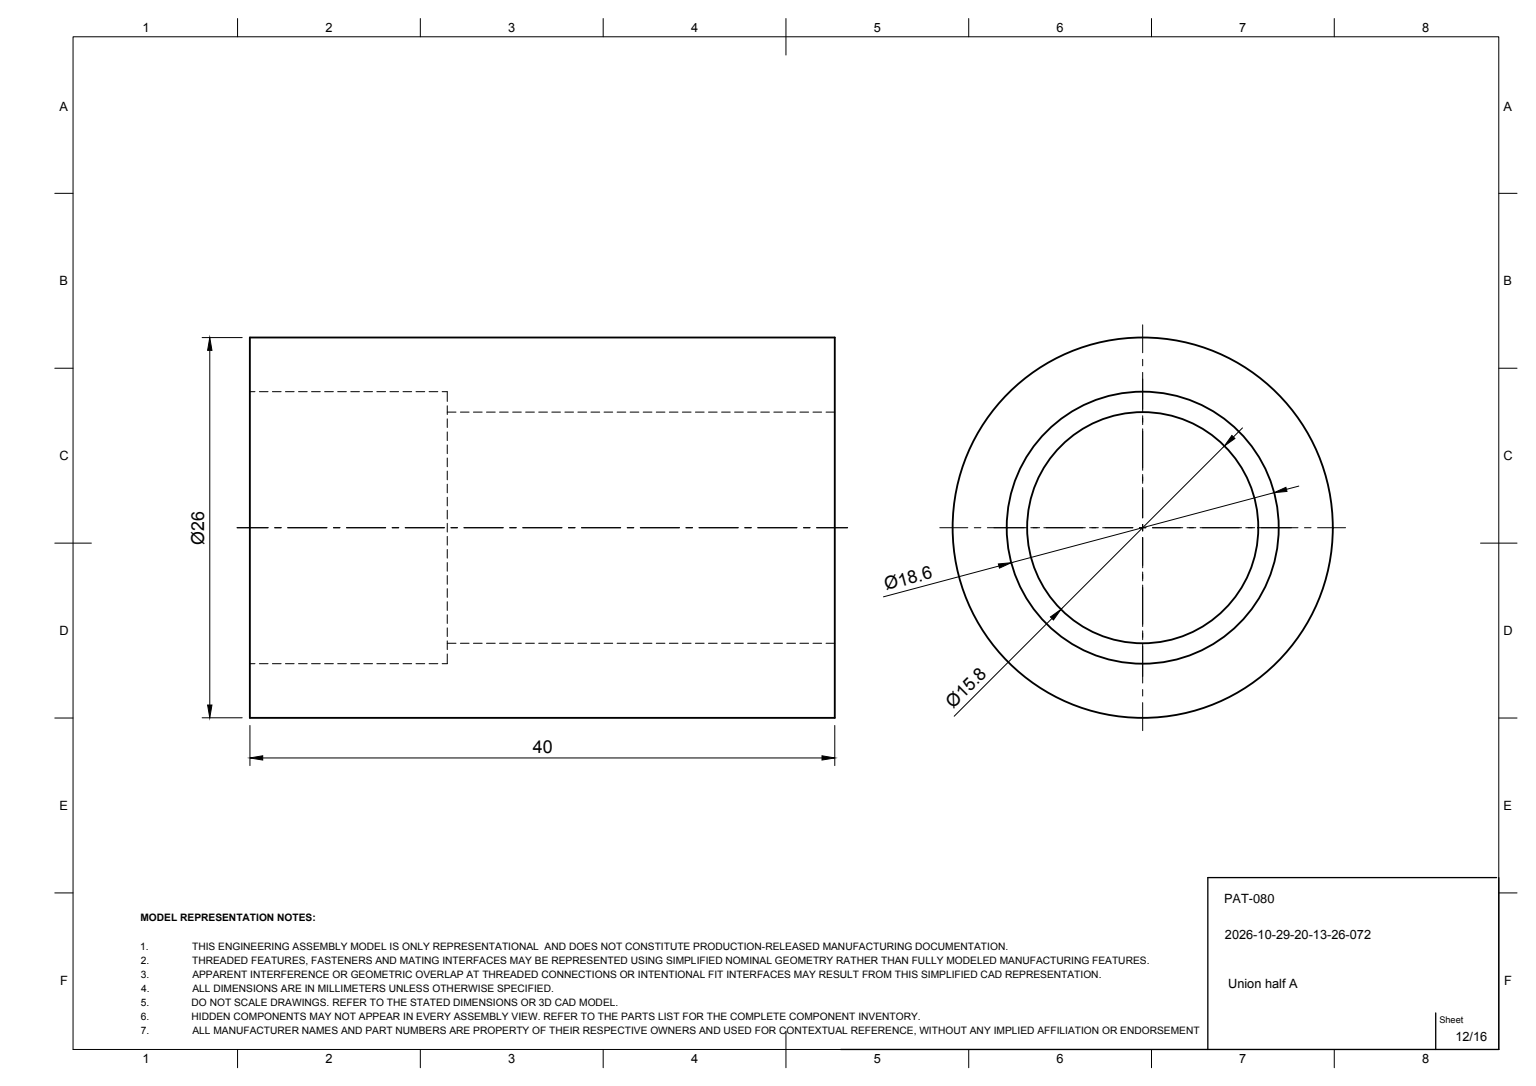
ISO-10303-21;
HEADER;
/* Generated by software containing ST-Developer
 * from STEP Tools, Inc. (www.steptools.com) 
 */

FILE_DESCRIPTION(
/* description */ ('PAT-080'),
/* implementation_level */ '2;1');

FILE_NAME(
/* name */ 'Union half A.step',
/* time_stamp */ '2026-10-29T20:13:47-07:00',
/* author */ (''),
/* organization */ (''),
/* preprocessor_version */ 'ST-DEVELOPER v20.2',
/* originating_system */ 'Autodesk Translation Framework v15.17.0.0',
/* authorisation */ '');

FILE_SCHEMA (('AUTOMOTIVE_DESIGN { 1 0 10303 214 3 1 1 }'));
ENDSEC;

DATA;
#10=MECHANICAL_DESIGN_GEOMETRIC_PRESENTATION_REPRESENTATION('',(#254),#6878);
#216=SHAPE_REPRESENTATION_RELATIONSHIP('SRR','None',#6972,#235);
#235=ADVANCED_BREP_SHAPE_REPRESENTATION('',(#273),#6867);
#254=STYLED_ITEM('',(#7143),#273);
#273=MANIFOLD_SOLID_BREP('Body1',#3870);
#312=FACE_BOUND('',#862,.T.);
#313=FACE_BOUND('',#863,.T.);
#314=FACE_BOUND('',#864,.T.);
#315=FACE_BOUND('',#865,.T.);
#316=FACE_BOUND('',#866,.T.);
#317=FACE_BOUND('',#871,.T.);
#318=FACE_BOUND('',#872,.T.);
#319=FACE_BOUND('',#873,.T.);
#320=FACE_BOUND('',#874,.T.);
#321=FACE_BOUND('',#875,.T.);
#322=FACE_BOUND('',#877,.T.);
#430=PLANE('',#4270);
#431=PLANE('',#4280);
#432=PLANE('',#4281);
#600=FACE_OUTER_BOUND('',#857,.T.);
#601=FACE_OUTER_BOUND('',#858,.T.);
#602=FACE_OUTER_BOUND('',#859,.T.);
#603=FACE_OUTER_BOUND('',#860,.T.);
#604=FACE_OUTER_BOUND('',#861,.T.);
#605=FACE_OUTER_BOUND('',#867,.T.);
#606=FACE_OUTER_BOUND('',#868,.T.);
#607=FACE_OUTER_BOUND('',#869,.T.);
#608=FACE_OUTER_BOUND('',#870,.T.);
#609=FACE_OUTER_BOUND('',#876,.T.);
#857=EDGE_LOOP('',(#3082,#3083,#3084,#3085));
#858=EDGE_LOOP('',(#3086,#3087,#3088,#3089));
#859=EDGE_LOOP('',(#3090,#3091,#3092,#3093));
#860=EDGE_LOOP('',(#3094,#3095,#3096,#3097));
#861=EDGE_LOOP('',(#3098));
#862=EDGE_LOOP('',(#3099));
#863=EDGE_LOOP('',(#3100));
#864=EDGE_LOOP('',(#3101));
#865=EDGE_LOOP('',(#3102));
#866=EDGE_LOOP('',(#3103));
#867=EDGE_LOOP('',(#3104,#3105,#3106,#3107));
#868=EDGE_LOOP('',(#3108,#3109,#3110,#3111));
#869=EDGE_LOOP('',(#3112,#3113,#3114,#3115));
#870=EDGE_LOOP('',(#3116));
#871=EDGE_LOOP('',(#3117));
#872=EDGE_LOOP('',(#3118));
#873=EDGE_LOOP('',(#3119));
#874=EDGE_LOOP('',(#3120));
#875=EDGE_LOOP('',(#3121));
#876=EDGE_LOOP('',(#3122));
#877=EDGE_LOOP('',(#3123));
#1211=LINE('',#6238,#1526);
#1212=LINE('',#6244,#1527);
#1213=LINE('',#6250,#1528);
#1214=LINE('',#6256,#1529);
#1215=LINE('',#6266,#1530);
#1216=LINE('',#6271,#1531);
#1217=LINE('',#6275,#1532);
#1526=VECTOR('',#5049,0.44);
#1527=VECTOR('',#5056,0.44);
#1528=VECTOR('',#5063,0.44);
#1529=VECTOR('',#5070,0.44);
#1530=VECTOR('',#5083,3.5);
#1531=VECTOR('',#5088,0.79);
#1532=VECTOR('',#5093,1.5);
#1712=CIRCLE('',#4259,0.44);
#1713=CIRCLE('',#4260,0.44);
#1714=CIRCLE('',#4262,0.44);
#1715=CIRCLE('',#4263,0.44);
#1716=CIRCLE('',#4265,0.44);
#1717=CIRCLE('',#4266,0.44);
#1718=CIRCLE('',#4268,0.44);
#1719=CIRCLE('',#4269,0.44);
#1720=CIRCLE('',#4271,3.5);
#1721=CIRCLE('',#4272,1.5);
#1722=CIRCLE('',#4274,3.5);
#1723=CIRCLE('',#4276,0.79);
#1724=CIRCLE('',#4277,0.79);
#1725=CIRCLE('',#4279,1.5);
#1968=VERTEX_POINT('',#6235);
#1969=VERTEX_POINT('',#6237);
#1970=VERTEX_POINT('',#6241);
#1971=VERTEX_POINT('',#6243);
#1972=VERTEX_POINT('',#6247);
#1973=VERTEX_POINT('',#6249);
#1974=VERTEX_POINT('',#6253);
#1975=VERTEX_POINT('',#6255);
#1976=VERTEX_POINT('',#6259);
#1977=VERTEX_POINT('',#6261);
#1978=VERTEX_POINT('',#6264);
#1979=VERTEX_POINT('',#6268);
#1980=VERTEX_POINT('',#6270);
#1981=VERTEX_POINT('',#6274);
#2364=EDGE_CURVE('',#1968,#1968,#1712,.T.);
#2365=EDGE_CURVE('',#1968,#1969,#1211,.T.);
#2366=EDGE_CURVE('',#1969,#1969,#1713,.T.);
#2367=EDGE_CURVE('',#1970,#1970,#1714,.T.);
#2368=EDGE_CURVE('',#1970,#1971,#1212,.T.);
#2369=EDGE_CURVE('',#1971,#1971,#1715,.T.);
#2370=EDGE_CURVE('',#1972,#1972,#1716,.T.);
#2371=EDGE_CURVE('',#1972,#1973,#1213,.T.);
#2372=EDGE_CURVE('',#1973,#1973,#1717,.T.);
#2373=EDGE_CURVE('',#1974,#1974,#1718,.T.);
#2374=EDGE_CURVE('',#1974,#1975,#1214,.T.);
#2375=EDGE_CURVE('',#1975,#1975,#1719,.T.);
#2376=EDGE_CURVE('',#1976,#1976,#1720,.T.);
#2377=EDGE_CURVE('',#1977,#1977,#1721,.T.);
#2378=EDGE_CURVE('',#1978,#1978,#1722,.T.);
#2379=EDGE_CURVE('',#1978,#1976,#1215,.T.);
#2380=EDGE_CURVE('',#1979,#1979,#1723,.T.);
#2381=EDGE_CURVE('',#1979,#1980,#1216,.T.);
#2382=EDGE_CURVE('',#1980,#1980,#1724,.T.);
#2383=EDGE_CURVE('',#1977,#1981,#1217,.T.);
#2384=EDGE_CURVE('',#1981,#1981,#1725,.T.);
#3082=ORIENTED_EDGE('',*,*,#2364,.F.);
#3083=ORIENTED_EDGE('',*,*,#2365,.T.);
#3084=ORIENTED_EDGE('',*,*,#2366,.F.);
#3085=ORIENTED_EDGE('',*,*,#2365,.F.);
#3086=ORIENTED_EDGE('',*,*,#2367,.F.);
#3087=ORIENTED_EDGE('',*,*,#2368,.T.);
#3088=ORIENTED_EDGE('',*,*,#2369,.F.);
#3089=ORIENTED_EDGE('',*,*,#2368,.F.);
#3090=ORIENTED_EDGE('',*,*,#2370,.F.);
#3091=ORIENTED_EDGE('',*,*,#2371,.T.);
#3092=ORIENTED_EDGE('',*,*,#2372,.F.);
#3093=ORIENTED_EDGE('',*,*,#2371,.F.);
#3094=ORIENTED_EDGE('',*,*,#2373,.F.);
#3095=ORIENTED_EDGE('',*,*,#2374,.T.);
#3096=ORIENTED_EDGE('',*,*,#2375,.F.);
#3097=ORIENTED_EDGE('',*,*,#2374,.F.);
#3098=ORIENTED_EDGE('',*,*,#2376,.F.);
#3099=ORIENTED_EDGE('',*,*,#2377,.F.);
#3100=ORIENTED_EDGE('',*,*,#2373,.T.);
#3101=ORIENTED_EDGE('',*,*,#2370,.T.);
#3102=ORIENTED_EDGE('',*,*,#2367,.T.);
#3103=ORIENTED_EDGE('',*,*,#2364,.T.);
#3104=ORIENTED_EDGE('',*,*,#2378,.F.);
#3105=ORIENTED_EDGE('',*,*,#2379,.T.);
#3106=ORIENTED_EDGE('',*,*,#2376,.T.);
#3107=ORIENTED_EDGE('',*,*,#2379,.F.);
#3108=ORIENTED_EDGE('',*,*,#2380,.F.);
#3109=ORIENTED_EDGE('',*,*,#2381,.T.);
#3110=ORIENTED_EDGE('',*,*,#2382,.T.);
#3111=ORIENTED_EDGE('',*,*,#2381,.F.);
#3112=ORIENTED_EDGE('',*,*,#2377,.T.);
#3113=ORIENTED_EDGE('',*,*,#2383,.T.);
#3114=ORIENTED_EDGE('',*,*,#2384,.T.);
#3115=ORIENTED_EDGE('',*,*,#2383,.F.);
#3116=ORIENTED_EDGE('',*,*,#2378,.T.);
#3117=ORIENTED_EDGE('',*,*,#2380,.T.);
#3118=ORIENTED_EDGE('',*,*,#2375,.T.);
#3119=ORIENTED_EDGE('',*,*,#2372,.T.);
#3120=ORIENTED_EDGE('',*,*,#2369,.T.);
#3121=ORIENTED_EDGE('',*,*,#2366,.T.);
#3122=ORIENTED_EDGE('',*,*,#2384,.F.);
#3123=ORIENTED_EDGE('',*,*,#2382,.F.);
#3597=CYLINDRICAL_SURFACE('',#4258,0.44);
#3598=CYLINDRICAL_SURFACE('',#4261,0.44);
#3599=CYLINDRICAL_SURFACE('',#4264,0.44);
#3600=CYLINDRICAL_SURFACE('',#4267,0.44);
#3601=CYLINDRICAL_SURFACE('',#4273,3.5);
#3602=CYLINDRICAL_SURFACE('',#4275,0.79);
#3603=CYLINDRICAL_SURFACE('',#4278,1.5);
#3736=ADVANCED_FACE('',(#600),#3597,.F.);
#3737=ADVANCED_FACE('',(#601),#3598,.F.);
#3738=ADVANCED_FACE('',(#602),#3599,.F.);
#3739=ADVANCED_FACE('',(#603),#3600,.F.);
#3740=ADVANCED_FACE('',(#604,#312,#313,#314,#315,#316),#430,.F.);
#3741=ADVANCED_FACE('',(#605),#3601,.T.);
#3742=ADVANCED_FACE('',(#606),#3602,.F.);
#3743=ADVANCED_FACE('',(#607),#3603,.T.);
#3744=ADVANCED_FACE('',(#608,#317,#318,#319,#320,#321),#431,.T.);
#3745=ADVANCED_FACE('',(#609,#322),#432,.F.);
#3870=CLOSED_SHELL('',(#3736,#3737,#3738,#3739,#3740,#3741,#3742,#3743,
#3744,#3745));
#4257=AXIS2_PLACEMENT_3D('',#6233,#5043,#5044);
#4258=AXIS2_PLACEMENT_3D('',#6234,#5045,#5046);
#4259=AXIS2_PLACEMENT_3D('',#6236,#5047,#5048);
#4260=AXIS2_PLACEMENT_3D('',#6239,#5050,#5051);
#4261=AXIS2_PLACEMENT_3D('',#6240,#5052,#5053);
#4262=AXIS2_PLACEMENT_3D('',#6242,#5054,#5055);
#4263=AXIS2_PLACEMENT_3D('',#6245,#5057,#5058);
#4264=AXIS2_PLACEMENT_3D('',#6246,#5059,#5060);
#4265=AXIS2_PLACEMENT_3D('',#6248,#5061,#5062);
#4266=AXIS2_PLACEMENT_3D('',#6251,#5064,#5065);
#4267=AXIS2_PLACEMENT_3D('',#6252,#5066,#5067);
#4268=AXIS2_PLACEMENT_3D('',#6254,#5068,#5069);
#4269=AXIS2_PLACEMENT_3D('',#6257,#5071,#5072);
#4270=AXIS2_PLACEMENT_3D('',#6258,#5073,#5074);
#4271=AXIS2_PLACEMENT_3D('',#6260,#5075,#5076);
#4272=AXIS2_PLACEMENT_3D('',#6262,#5077,#5078);
#4273=AXIS2_PLACEMENT_3D('',#6263,#5079,#5080);
#4274=AXIS2_PLACEMENT_3D('',#6265,#5081,#5082);
#4275=AXIS2_PLACEMENT_3D('',#6267,#5084,#5085);
#4276=AXIS2_PLACEMENT_3D('',#6269,#5086,#5087);
#4277=AXIS2_PLACEMENT_3D('',#6272,#5089,#5090);
#4278=AXIS2_PLACEMENT_3D('',#6273,#5091,#5092);
#4279=AXIS2_PLACEMENT_3D('',#6276,#5094,#5095);
#4280=AXIS2_PLACEMENT_3D('',#6277,#5096,#5097);
#4281=AXIS2_PLACEMENT_3D('',#6278,#5098,#5099);
#5043=DIRECTION('axis',(0.,0.,1.));
#5044=DIRECTION('refdir',(1.,0.,0.));
#5045=DIRECTION('center_axis',(1.,0.,0.));
#5046=DIRECTION('ref_axis',(0.,0.,-1.));
#5047=DIRECTION('center_axis',(1.,0.,0.));
#5048=DIRECTION('ref_axis',(0.,0.,-1.));
#5049=DIRECTION('',(1.,0.,0.));
#5050=DIRECTION('center_axis',(-1.,0.,0.));
#5051=DIRECTION('ref_axis',(0.,0.,-1.));
#5052=DIRECTION('center_axis',(1.,0.,0.));
#5053=DIRECTION('ref_axis',(0.,0.,-1.));
#5054=DIRECTION('center_axis',(1.,0.,0.));
#5055=DIRECTION('ref_axis',(0.,0.,-1.));
#5056=DIRECTION('',(1.,0.,0.));
#5057=DIRECTION('center_axis',(-1.,0.,0.));
#5058=DIRECTION('ref_axis',(0.,0.,-1.));
#5059=DIRECTION('center_axis',(1.,0.,0.));
#5060=DIRECTION('ref_axis',(0.,0.,-1.));
#5061=DIRECTION('center_axis',(1.,0.,0.));
#5062=DIRECTION('ref_axis',(0.,0.,-1.));
#5063=DIRECTION('',(1.,0.,0.));
#5064=DIRECTION('center_axis',(-1.,0.,0.));
#5065=DIRECTION('ref_axis',(0.,0.,-1.));
#5066=DIRECTION('center_axis',(1.,0.,0.));
#5067=DIRECTION('ref_axis',(0.,0.,-1.));
#5068=DIRECTION('center_axis',(1.,0.,0.));
#5069=DIRECTION('ref_axis',(0.,0.,-1.));
#5070=DIRECTION('',(1.,0.,0.));
#5071=DIRECTION('center_axis',(-1.,0.,0.));
#5072=DIRECTION('ref_axis',(0.,0.,-1.));
#5073=DIRECTION('center_axis',(1.,0.,0.));
#5074=DIRECTION('ref_axis',(0.,0.,-1.));
#5075=DIRECTION('center_axis',(1.,0.,0.));
#5076=DIRECTION('ref_axis',(0.,0.,-1.));
#5077=DIRECTION('center_axis',(-1.,0.,0.));
#5078=DIRECTION('ref_axis',(0.,0.,-1.));
#5079=DIRECTION('center_axis',(1.,0.,0.));
#5080=DIRECTION('ref_axis',(0.,0.,-1.));
#5081=DIRECTION('center_axis',(1.,0.,0.));
#5082=DIRECTION('ref_axis',(0.,0.,-1.));
#5083=DIRECTION('',(-1.,0.,0.));
#5084=DIRECTION('center_axis',(1.,0.,0.));
#5085=DIRECTION('ref_axis',(0.,0.,-1.));
#5086=DIRECTION('center_axis',(-1.,0.,0.));
#5087=DIRECTION('ref_axis',(0.,0.,-1.));
#5088=DIRECTION('',(-1.,0.,0.));
#5089=DIRECTION('center_axis',(-1.,0.,0.));
#5090=DIRECTION('ref_axis',(0.,0.,-1.));
#5091=DIRECTION('center_axis',(1.,0.,0.));
#5092=DIRECTION('ref_axis',(0.,0.,-1.));
#5093=DIRECTION('',(-1.,0.,0.));
#5094=DIRECTION('center_axis',(1.,0.,0.));
#5095=DIRECTION('ref_axis',(0.,0.,-1.));
#5096=DIRECTION('center_axis',(1.,0.,0.));
#5097=DIRECTION('ref_axis',(0.,0.,-1.));
#5098=DIRECTION('center_axis',(1.,0.,0.));
#5099=DIRECTION('ref_axis',(0.,0.,-1.));
#6233=CARTESIAN_POINT('',(0.,0.,0.));
#6234=CARTESIAN_POINT('Origin',(-0.9,-1.90918830920368,4.09081169079632));
#6235=CARTESIAN_POINT('',(-0.8,-1.90918830920368,4.53081169079632));
#6236=CARTESIAN_POINT('Origin',(-0.8,-1.90918830920368,4.09081169079632));
#6237=CARTESIAN_POINT('',(-0.1,-1.90918830920368,4.53081169079632));
#6238=CARTESIAN_POINT('',(-0.9,-1.90918830920368,4.53081169079632));
#6239=CARTESIAN_POINT('Origin',(-0.1,-1.90918830920368,4.09081169079632));
#6240=CARTESIAN_POINT('Origin',(-0.9,-1.90918830920368,7.90918830920368));
#6241=CARTESIAN_POINT('',(-0.8,-1.90918830920368,8.34918830920368));
#6242=CARTESIAN_POINT('Origin',(-0.8,-1.90918830920368,7.90918830920368));
#6243=CARTESIAN_POINT('',(-0.1,-1.90918830920368,8.34918830920368));
#6244=CARTESIAN_POINT('',(-0.9,-1.90918830920368,8.34918830920368));
#6245=CARTESIAN_POINT('Origin',(-0.1,-1.90918830920368,7.90918830920368));
#6246=CARTESIAN_POINT('Origin',(-0.9,1.90918830920368,7.90918830920368));
#6247=CARTESIAN_POINT('',(-0.8,1.90918830920368,8.34918830920368));
#6248=CARTESIAN_POINT('Origin',(-0.8,1.90918830920368,7.90918830920368));
#6249=CARTESIAN_POINT('',(-0.1,1.90918830920368,8.34918830920368));
#6250=CARTESIAN_POINT('',(-0.9,1.90918830920368,8.34918830920368));
#6251=CARTESIAN_POINT('Origin',(-0.1,1.90918830920368,7.90918830920368));
#6252=CARTESIAN_POINT('Origin',(-0.9,1.90918830920368,4.09081169079632));
#6253=CARTESIAN_POINT('',(-0.8,1.90918830920368,4.53081169079632));
#6254=CARTESIAN_POINT('Origin',(-0.8,1.90918830920368,4.09081169079632));
#6255=CARTESIAN_POINT('',(-0.1,1.90918830920368,4.53081169079632));
#6256=CARTESIAN_POINT('',(-0.9,1.90918830920368,4.53081169079632));
#6257=CARTESIAN_POINT('Origin',(-0.1,1.90918830920368,4.09081169079632));
#6258=CARTESIAN_POINT('Origin',(-0.8,0.,6.));
#6259=CARTESIAN_POINT('',(-0.8,-4.28626379701574E-16,9.5));
#6260=CARTESIAN_POINT('Origin',(-0.8,0.,6.));
#6261=CARTESIAN_POINT('',(-0.8,1.83697019872103E-16,7.5));
#6262=CARTESIAN_POINT('Origin',(-0.8,0.,6.));
#6263=CARTESIAN_POINT('Origin',(-0.8,0.,6.));
#6264=CARTESIAN_POINT('',(-0.1,-4.28626379701574E-16,9.5));
#6265=CARTESIAN_POINT('Origin',(-0.1,0.,6.));
#6266=CARTESIAN_POINT('',(-0.8,-4.28626379701574E-16,9.5));
#6267=CARTESIAN_POINT('Origin',(-2.8,0.,6.));
#6268=CARTESIAN_POINT('',(-0.1,-9.67470971326409E-17,6.79));
#6269=CARTESIAN_POINT('Origin',(-0.1,0.,6.));
#6270=CARTESIAN_POINT('',(-2.8,-9.67470971326409E-17,6.79));
#6271=CARTESIAN_POINT('',(-2.8,-9.67470971326409E-17,6.79));
#6272=CARTESIAN_POINT('Origin',(-2.8,0.,6.));
#6273=CARTESIAN_POINT('Origin',(-2.8,0.,6.));
#6274=CARTESIAN_POINT('',(-2.8,-1.83697019872103E-16,7.5));
#6275=CARTESIAN_POINT('',(-2.8,-1.83697019872103E-16,7.5));
#6276=CARTESIAN_POINT('Origin',(-2.8,0.,6.));
#6277=CARTESIAN_POINT('Origin',(-0.1,0.,6.));
#6278=CARTESIAN_POINT('Origin',(-2.8,0.,6.));
#6846=UNCERTAINTY_MEASURE_WITH_UNIT(LENGTH_MEASURE(0.001),#6879,
'DISTANCE_ACCURACY_VALUE',
'Maximum model space distance between geometric entities at asserted c
onnectivities');
#6857=UNCERTAINTY_MEASURE_WITH_UNIT(LENGTH_MEASURE(0.001),#6879,
'DISTANCE_ACCURACY_VALUE',
'Maximum model space distance between geometric entities at asserted c
onnectivities');
#6867=(
GEOMETRIC_REPRESENTATION_CONTEXT(3)
GLOBAL_UNCERTAINTY_ASSIGNED_CONTEXT((#6846))
GLOBAL_UNIT_ASSIGNED_CONTEXT((#6879,#6881,#6882))
REPRESENTATION_CONTEXT('','3D')
);
#6878=(
GEOMETRIC_REPRESENTATION_CONTEXT(3)
GLOBAL_UNCERTAINTY_ASSIGNED_CONTEXT((#6857))
GLOBAL_UNIT_ASSIGNED_CONTEXT((#6879,#6881,#6882))
REPRESENTATION_CONTEXT('','3D')
);
#6879=(
LENGTH_UNIT()
NAMED_UNIT(*)
SI_UNIT(.CENTI.,.METRE.)
);
#6881=(
NAMED_UNIT(*)
PLANE_ANGLE_UNIT()
SI_UNIT($,.RADIAN.)
);
#6882=(
NAMED_UNIT(*)
SI_UNIT($,.STERADIAN.)
SOLID_ANGLE_UNIT()
);
#6892=SHAPE_DEFINITION_REPRESENTATION(#6912,#6972);
#6912=PRODUCT_DEFINITION_SHAPE('',$,#6993);
#6972=SHAPE_REPRESENTATION('',(#4257),#6867);
#6983=PRODUCT_DEFINITION_CONTEXT('part definition',#7045,'design');
#6993=PRODUCT_DEFINITION('Union half A','Union half A',#7013,
#6983);
#7013=PRODUCT_DEFINITION_FORMATION('',$,#7056);
#7045=APPLICATION_CONTEXT(
'Core Data for Automotive Mechanical Design Process');
#7046=PRODUCT_CONTEXT('part definition',#7045,'mechanical');
#7056=PRODUCT('Union half A','Union half A','Union half A',
(#7046));
#7137=COLOUR_RGB('Off White',0.89,0.88,0.83);
#7138=FILL_AREA_STYLE_COLOUR('',#7137);
#7139=FILL_AREA_STYLE('',(#7138));
#7140=SURFACE_STYLE_FILL_AREA(#7139);
#7141=SURFACE_SIDE_STYLE('',(#7140));
#7142=SURFACE_STYLE_USAGE(.BOTH.,#7141);
#7143=PRESENTATION_STYLE_ASSIGNMENT((#7142));
ENDSEC;
END-ISO-10303-21;
